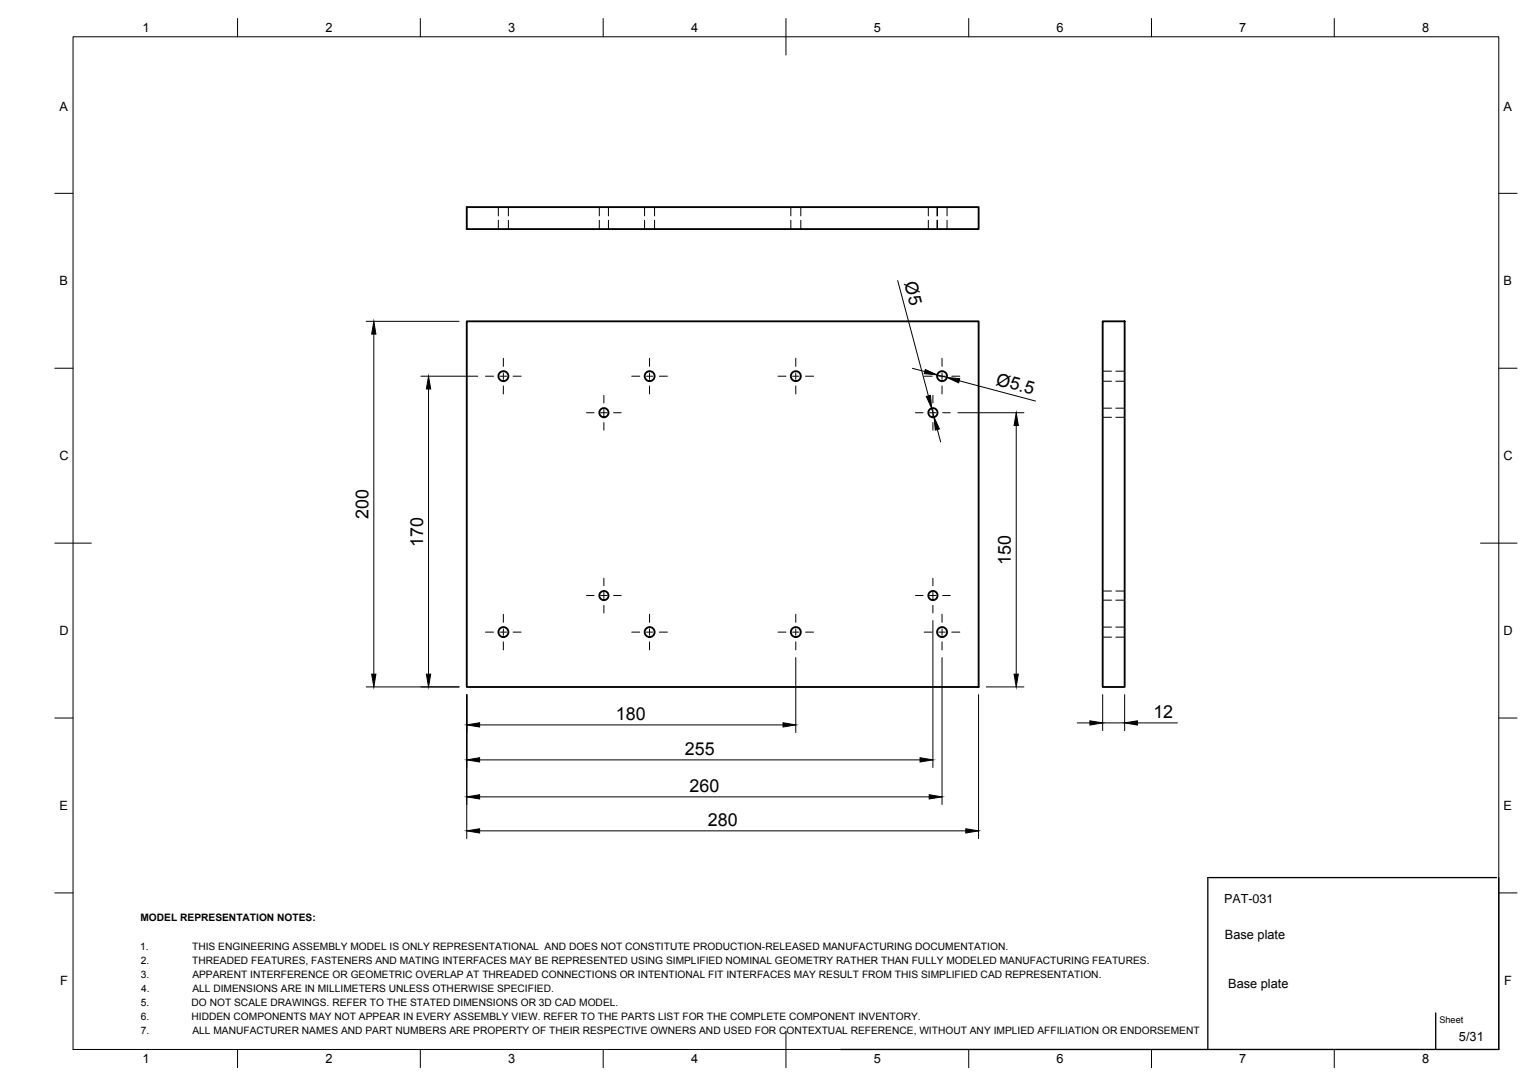
ISO-10303-21;
HEADER;
/* Generated by software containing ST-Developer
 * from STEP Tools, Inc. (www.steptools.com) 
 */

FILE_DESCRIPTION(
/* description */ ('Double-row support with tensioned shaft'),
/* implementation_level */ '2;1');

FILE_NAME(
/* name */ 'Base plate.step',
/* time_stamp */ '2026-10-27T10:50:35-07:00',
/* author */ (''),
/* organization */ (''),
/* preprocessor_version */ 'ST-DEVELOPER v20.2',
/* originating_system */ 'Autodesk Translation Framework v15.17.0.0',
/* authorisation */ '');

FILE_SCHEMA (('AUTOMOTIVE_DESIGN { 1 0 10303 214 3 1 1 }'));
ENDSEC;

DATA;
#10=MECHANICAL_DESIGN_GEOMETRIC_PRESENTATION_REPRESENTATION('',(#479),#11559);
#415=SHAPE_REPRESENTATION_RELATIONSHIP('SRR','None',#11723,#447);
#447=ADVANCED_BREP_SHAPE_REPRESENTATION('',(#512),#11525);
#479=STYLED_ITEM('',(#11946),#512);
#512=MANIFOLD_SOLID_BREP('Body1',#6324);
#542=FACE_BOUND('',#1278,.T.);
#543=FACE_BOUND('',#1279,.T.);
#544=FACE_BOUND('',#1280,.T.);
#545=FACE_BOUND('',#1281,.T.);
#546=FACE_BOUND('',#1282,.T.);
#547=FACE_BOUND('',#1283,.T.);
#548=FACE_BOUND('',#1284,.T.);
#549=FACE_BOUND('',#1285,.T.);
#550=FACE_BOUND('',#1286,.T.);
#551=FACE_BOUND('',#1287,.T.);
#552=FACE_BOUND('',#1288,.T.);
#553=FACE_BOUND('',#1289,.T.);
#554=FACE_BOUND('',#1291,.T.);
#555=FACE_BOUND('',#1292,.T.);
#556=FACE_BOUND('',#1293,.T.);
#557=FACE_BOUND('',#1294,.T.);
#558=FACE_BOUND('',#1295,.T.);
#559=FACE_BOUND('',#1296,.T.);
#560=FACE_BOUND('',#1297,.T.);
#561=FACE_BOUND('',#1298,.T.);
#562=FACE_BOUND('',#1299,.T.);
#563=FACE_BOUND('',#1300,.T.);
#564=FACE_BOUND('',#1301,.T.);
#565=FACE_BOUND('',#1302,.T.);
#679=PLANE('',#6752);
#680=PLANE('',#6753);
#681=PLANE('',#6754);
#682=PLANE('',#6755);
#683=PLANE('',#6756);
#684=PLANE('',#6757);
#917=FACE_OUTER_BOUND('',#1261,.T.);
#918=FACE_OUTER_BOUND('',#1262,.T.);
#919=FACE_OUTER_BOUND('',#1263,.T.);
#920=FACE_OUTER_BOUND('',#1264,.T.);
#921=FACE_OUTER_BOUND('',#1265,.T.);
#922=FACE_OUTER_BOUND('',#1266,.T.);
#923=FACE_OUTER_BOUND('',#1267,.T.);
#924=FACE_OUTER_BOUND('',#1268,.T.);
#925=FACE_OUTER_BOUND('',#1269,.T.);
#926=FACE_OUTER_BOUND('',#1270,.T.);
#927=FACE_OUTER_BOUND('',#1271,.T.);
#928=FACE_OUTER_BOUND('',#1272,.T.);
#929=FACE_OUTER_BOUND('',#1273,.T.);
#930=FACE_OUTER_BOUND('',#1274,.T.);
#931=FACE_OUTER_BOUND('',#1275,.T.);
#932=FACE_OUTER_BOUND('',#1276,.T.);
#933=FACE_OUTER_BOUND('',#1277,.T.);
#934=FACE_OUTER_BOUND('',#1290,.T.);
#1261=EDGE_LOOP('',(#4330,#4331,#4332,#4333));
#1262=EDGE_LOOP('',(#4334,#4335,#4336,#4337));
#1263=EDGE_LOOP('',(#4338,#4339,#4340,#4341));
#1264=EDGE_LOOP('',(#4342,#4343,#4344,#4345));
#1265=EDGE_LOOP('',(#4346,#4347,#4348,#4349));
#1266=EDGE_LOOP('',(#4350,#4351,#4352,#4353));
#1267=EDGE_LOOP('',(#4354,#4355,#4356,#4357));
#1268=EDGE_LOOP('',(#4358,#4359,#4360,#4361));
#1269=EDGE_LOOP('',(#4362,#4363,#4364,#4365));
#1270=EDGE_LOOP('',(#4366,#4367,#4368,#4369));
#1271=EDGE_LOOP('',(#4370,#4371,#4372,#4373));
#1272=EDGE_LOOP('',(#4374,#4375,#4376,#4377));
#1273=EDGE_LOOP('',(#4378,#4379,#4380,#4381));
#1274=EDGE_LOOP('',(#4382,#4383,#4384,#4385));
#1275=EDGE_LOOP('',(#4386,#4387,#4388,#4389));
#1276=EDGE_LOOP('',(#4390,#4391,#4392,#4393));
#1277=EDGE_LOOP('',(#4394,#4395,#4396,#4397));
#1278=EDGE_LOOP('',(#4398));
#1279=EDGE_LOOP('',(#4399));
#1280=EDGE_LOOP('',(#4400));
#1281=EDGE_LOOP('',(#4401));
#1282=EDGE_LOOP('',(#4402));
#1283=EDGE_LOOP('',(#4403));
#1284=EDGE_LOOP('',(#4404));
#1285=EDGE_LOOP('',(#4405));
#1286=EDGE_LOOP('',(#4406));
#1287=EDGE_LOOP('',(#4407));
#1288=EDGE_LOOP('',(#4408));
#1289=EDGE_LOOP('',(#4409));
#1290=EDGE_LOOP('',(#4410,#4411,#4412,#4413));
#1291=EDGE_LOOP('',(#4414));
#1292=EDGE_LOOP('',(#4415));
#1293=EDGE_LOOP('',(#4416));
#1294=EDGE_LOOP('',(#4417));
#1295=EDGE_LOOP('',(#4418));
#1296=EDGE_LOOP('',(#4419));
#1297=EDGE_LOOP('',(#4420));
#1298=EDGE_LOOP('',(#4421));
#1299=EDGE_LOOP('',(#4422));
#1300=EDGE_LOOP('',(#4423));
#1301=EDGE_LOOP('',(#4424));
#1302=EDGE_LOOP('',(#4425));
#1742=LINE('',#9241,#2289);
#1743=LINE('',#9247,#2290);
#1744=LINE('',#9253,#2291);
#1745=LINE('',#9259,#2292);
#1746=LINE('',#9265,#2293);
#1747=LINE('',#9271,#2294);
#1748=LINE('',#9277,#2295);
#1749=LINE('',#9283,#2296);
#1750=LINE('',#9289,#2297);
#1751=LINE('',#9295,#2298);
#1752=LINE('',#9301,#2299);
#1753=LINE('',#9307,#2300);
#1754=LINE('',#9312,#2301);
#1755=LINE('',#9314,#2302);
#1756=LINE('',#9316,#2303);
#1757=LINE('',#9317,#2304);
#1758=LINE('',#9320,#2305);
#1759=LINE('',#9322,#2306);
#1760=LINE('',#9323,#2307);
#1761=LINE('',#9326,#2308);
#1762=LINE('',#9328,#2309);
#1763=LINE('',#9329,#2310);
#1764=LINE('',#9331,#2311);
#1765=LINE('',#9332,#2312);
#2289=VECTOR('',#7381,0.25);
#2290=VECTOR('',#7388,0.25);
#2291=VECTOR('',#7395,0.25);
#2292=VECTOR('',#7402,0.25);
#2293=VECTOR('',#7409,0.275);
#2294=VECTOR('',#7416,0.275);
#2295=VECTOR('',#7423,0.275);
#2296=VECTOR('',#7430,0.275);
#2297=VECTOR('',#7437,0.275);
#2298=VECTOR('',#7444,0.275);
#2299=VECTOR('',#7451,0.275);
#2300=VECTOR('',#7458,0.275);
#2301=VECTOR('',#7463,1.);
#2302=VECTOR('',#7464,1.);
#2303=VECTOR('',#7465,1.);
#2304=VECTOR('',#7466,1.);
#2305=VECTOR('',#7469,1.);
#2306=VECTOR('',#7470,1.);
#2307=VECTOR('',#7471,1.);
#2308=VECTOR('',#7474,1.);
#2309=VECTOR('',#7475,1.);
#2310=VECTOR('',#7476,1.);
#2311=VECTOR('',#7479,1.);
#2312=VECTOR('',#7480,1.);
#2836=CIRCLE('',#6717,0.25);
#2837=CIRCLE('',#6718,0.25);
#2838=CIRCLE('',#6720,0.25);
#2839=CIRCLE('',#6721,0.25);
#2840=CIRCLE('',#6723,0.25);
#2841=CIRCLE('',#6724,0.25);
#2842=CIRCLE('',#6726,0.25);
#2843=CIRCLE('',#6727,0.25);
#2844=CIRCLE('',#6729,0.275);
#2845=CIRCLE('',#6730,0.275);
#2846=CIRCLE('',#6732,0.275);
#2847=CIRCLE('',#6733,0.275);
#2848=CIRCLE('',#6735,0.275);
#2849=CIRCLE('',#6736,0.275);
#2850=CIRCLE('',#6738,0.275);
#2851=CIRCLE('',#6739,0.275);
#2852=CIRCLE('',#6741,0.275);
#2853=CIRCLE('',#6742,0.275);
#2854=CIRCLE('',#6744,0.275);
#2855=CIRCLE('',#6745,0.275);
#2856=CIRCLE('',#6747,0.275);
#2857=CIRCLE('',#6748,0.275);
#2858=CIRCLE('',#6750,0.275);
#2859=CIRCLE('',#6751,0.275);
#3027=VERTEX_POINT('',#9238);
#3028=VERTEX_POINT('',#9240);
#3029=VERTEX_POINT('',#9244);
#3030=VERTEX_POINT('',#9246);
#3031=VERTEX_POINT('',#9250);
#3032=VERTEX_POINT('',#9252);
#3033=VERTEX_POINT('',#9256);
#3034=VERTEX_POINT('',#9258);
#3035=VERTEX_POINT('',#9262);
#3036=VERTEX_POINT('',#9264);
#3037=VERTEX_POINT('',#9268);
#3038=VERTEX_POINT('',#9270);
#3039=VERTEX_POINT('',#9274);
#3040=VERTEX_POINT('',#9276);
#3041=VERTEX_POINT('',#9280);
#3042=VERTEX_POINT('',#9282);
#3043=VERTEX_POINT('',#9286);
#3044=VERTEX_POINT('',#9288);
#3045=VERTEX_POINT('',#9292);
#3046=VERTEX_POINT('',#9294);
#3047=VERTEX_POINT('',#9298);
#3048=VERTEX_POINT('',#9300);
#3049=VERTEX_POINT('',#9304);
#3050=VERTEX_POINT('',#9306);
#3051=VERTEX_POINT('',#9310);
#3052=VERTEX_POINT('',#9311);
#3053=VERTEX_POINT('',#9313);
#3054=VERTEX_POINT('',#9315);
#3055=VERTEX_POINT('',#9319);
#3056=VERTEX_POINT('',#9321);
#3057=VERTEX_POINT('',#9325);
#3058=VERTEX_POINT('',#9327);
#3550=EDGE_CURVE('',#3027,#3027,#2836,.T.);
#3551=EDGE_CURVE('',#3027,#3028,#1742,.T.);
#3552=EDGE_CURVE('',#3028,#3028,#2837,.T.);
#3553=EDGE_CURVE('',#3029,#3029,#2838,.T.);
#3554=EDGE_CURVE('',#3029,#3030,#1743,.T.);
#3555=EDGE_CURVE('',#3030,#3030,#2839,.T.);
#3556=EDGE_CURVE('',#3031,#3031,#2840,.T.);
#3557=EDGE_CURVE('',#3031,#3032,#1744,.T.);
#3558=EDGE_CURVE('',#3032,#3032,#2841,.T.);
#3559=EDGE_CURVE('',#3033,#3033,#2842,.T.);
#3560=EDGE_CURVE('',#3033,#3034,#1745,.T.);
#3561=EDGE_CURVE('',#3034,#3034,#2843,.T.);
#3562=EDGE_CURVE('',#3035,#3035,#2844,.T.);
#3563=EDGE_CURVE('',#3035,#3036,#1746,.T.);
#3564=EDGE_CURVE('',#3036,#3036,#2845,.T.);
#3565=EDGE_CURVE('',#3037,#3037,#2846,.T.);
#3566=EDGE_CURVE('',#3037,#3038,#1747,.T.);
#3567=EDGE_CURVE('',#3038,#3038,#2847,.T.);
#3568=EDGE_CURVE('',#3039,#3039,#2848,.T.);
#3569=EDGE_CURVE('',#3039,#3040,#1748,.T.);
#3570=EDGE_CURVE('',#3040,#3040,#2849,.T.);
#3571=EDGE_CURVE('',#3041,#3041,#2850,.T.);
#3572=EDGE_CURVE('',#3041,#3042,#1749,.T.);
#3573=EDGE_CURVE('',#3042,#3042,#2851,.T.);
#3574=EDGE_CURVE('',#3043,#3043,#2852,.T.);
#3575=EDGE_CURVE('',#3043,#3044,#1750,.T.);
#3576=EDGE_CURVE('',#3044,#3044,#2853,.T.);
#3577=EDGE_CURVE('',#3045,#3045,#2854,.T.);
#3578=EDGE_CURVE('',#3045,#3046,#1751,.T.);
#3579=EDGE_CURVE('',#3046,#3046,#2855,.T.);
#3580=EDGE_CURVE('',#3047,#3047,#2856,.T.);
#3581=EDGE_CURVE('',#3047,#3048,#1752,.T.);
#3582=EDGE_CURVE('',#3048,#3048,#2857,.T.);
#3583=EDGE_CURVE('',#3049,#3049,#2858,.T.);
#3584=EDGE_CURVE('',#3049,#3050,#1753,.T.);
#3585=EDGE_CURVE('',#3050,#3050,#2859,.T.);
#3586=EDGE_CURVE('',#3051,#3052,#1754,.T.);
#3587=EDGE_CURVE('',#3052,#3053,#1755,.T.);
#3588=EDGE_CURVE('',#3054,#3053,#1756,.T.);
#3589=EDGE_CURVE('',#3051,#3054,#1757,.T.);
#3590=EDGE_CURVE('',#3055,#3051,#1758,.T.);
#3591=EDGE_CURVE('',#3056,#3054,#1759,.T.);
#3592=EDGE_CURVE('',#3055,#3056,#1760,.T.);
#3593=EDGE_CURVE('',#3057,#3055,#1761,.T.);
#3594=EDGE_CURVE('',#3058,#3056,#1762,.T.);
#3595=EDGE_CURVE('',#3057,#3058,#1763,.T.);
#3596=EDGE_CURVE('',#3052,#3057,#1764,.T.);
#3597=EDGE_CURVE('',#3053,#3058,#1765,.T.);
#4330=ORIENTED_EDGE('',*,*,#3550,.F.);
#4331=ORIENTED_EDGE('',*,*,#3551,.T.);
#4332=ORIENTED_EDGE('',*,*,#3552,.F.);
#4333=ORIENTED_EDGE('',*,*,#3551,.F.);
#4334=ORIENTED_EDGE('',*,*,#3553,.F.);
#4335=ORIENTED_EDGE('',*,*,#3554,.T.);
#4336=ORIENTED_EDGE('',*,*,#3555,.F.);
#4337=ORIENTED_EDGE('',*,*,#3554,.F.);
#4338=ORIENTED_EDGE('',*,*,#3556,.F.);
#4339=ORIENTED_EDGE('',*,*,#3557,.T.);
#4340=ORIENTED_EDGE('',*,*,#3558,.F.);
#4341=ORIENTED_EDGE('',*,*,#3557,.F.);
#4342=ORIENTED_EDGE('',*,*,#3559,.F.);
#4343=ORIENTED_EDGE('',*,*,#3560,.T.);
#4344=ORIENTED_EDGE('',*,*,#3561,.F.);
#4345=ORIENTED_EDGE('',*,*,#3560,.F.);
#4346=ORIENTED_EDGE('',*,*,#3562,.F.);
#4347=ORIENTED_EDGE('',*,*,#3563,.T.);
#4348=ORIENTED_EDGE('',*,*,#3564,.F.);
#4349=ORIENTED_EDGE('',*,*,#3563,.F.);
#4350=ORIENTED_EDGE('',*,*,#3565,.F.);
#4351=ORIENTED_EDGE('',*,*,#3566,.T.);
#4352=ORIENTED_EDGE('',*,*,#3567,.F.);
#4353=ORIENTED_EDGE('',*,*,#3566,.F.);
#4354=ORIENTED_EDGE('',*,*,#3568,.F.);
#4355=ORIENTED_EDGE('',*,*,#3569,.T.);
#4356=ORIENTED_EDGE('',*,*,#3570,.F.);
#4357=ORIENTED_EDGE('',*,*,#3569,.F.);
#4358=ORIENTED_EDGE('',*,*,#3571,.F.);
#4359=ORIENTED_EDGE('',*,*,#3572,.T.);
#4360=ORIENTED_EDGE('',*,*,#3573,.F.);
#4361=ORIENTED_EDGE('',*,*,#3572,.F.);
#4362=ORIENTED_EDGE('',*,*,#3574,.F.);
#4363=ORIENTED_EDGE('',*,*,#3575,.T.);
#4364=ORIENTED_EDGE('',*,*,#3576,.F.);
#4365=ORIENTED_EDGE('',*,*,#3575,.F.);
#4366=ORIENTED_EDGE('',*,*,#3577,.F.);
#4367=ORIENTED_EDGE('',*,*,#3578,.T.);
#4368=ORIENTED_EDGE('',*,*,#3579,.F.);
#4369=ORIENTED_EDGE('',*,*,#3578,.F.);
#4370=ORIENTED_EDGE('',*,*,#3580,.F.);
#4371=ORIENTED_EDGE('',*,*,#3581,.T.);
#4372=ORIENTED_EDGE('',*,*,#3582,.F.);
#4373=ORIENTED_EDGE('',*,*,#3581,.F.);
#4374=ORIENTED_EDGE('',*,*,#3583,.F.);
#4375=ORIENTED_EDGE('',*,*,#3584,.T.);
#4376=ORIENTED_EDGE('',*,*,#3585,.F.);
#4377=ORIENTED_EDGE('',*,*,#3584,.F.);
#4378=ORIENTED_EDGE('',*,*,#3586,.T.);
#4379=ORIENTED_EDGE('',*,*,#3587,.T.);
#4380=ORIENTED_EDGE('',*,*,#3588,.F.);
#4381=ORIENTED_EDGE('',*,*,#3589,.F.);
#4382=ORIENTED_EDGE('',*,*,#3590,.T.);
#4383=ORIENTED_EDGE('',*,*,#3589,.T.);
#4384=ORIENTED_EDGE('',*,*,#3591,.F.);
#4385=ORIENTED_EDGE('',*,*,#3592,.F.);
#4386=ORIENTED_EDGE('',*,*,#3593,.T.);
#4387=ORIENTED_EDGE('',*,*,#3592,.T.);
#4388=ORIENTED_EDGE('',*,*,#3594,.F.);
#4389=ORIENTED_EDGE('',*,*,#3595,.F.);
#4390=ORIENTED_EDGE('',*,*,#3596,.T.);
#4391=ORIENTED_EDGE('',*,*,#3595,.T.);
#4392=ORIENTED_EDGE('',*,*,#3597,.F.);
#4393=ORIENTED_EDGE('',*,*,#3587,.F.);
#4394=ORIENTED_EDGE('',*,*,#3597,.T.);
#4395=ORIENTED_EDGE('',*,*,#3594,.T.);
#4396=ORIENTED_EDGE('',*,*,#3591,.T.);
#4397=ORIENTED_EDGE('',*,*,#3588,.T.);
#4398=ORIENTED_EDGE('',*,*,#3558,.T.);
#4399=ORIENTED_EDGE('',*,*,#3561,.T.);
#4400=ORIENTED_EDGE('',*,*,#3585,.T.);
#4401=ORIENTED_EDGE('',*,*,#3582,.T.);
#4402=ORIENTED_EDGE('',*,*,#3579,.T.);
#4403=ORIENTED_EDGE('',*,*,#3576,.T.);
#4404=ORIENTED_EDGE('',*,*,#3573,.T.);
#4405=ORIENTED_EDGE('',*,*,#3570,.T.);
#4406=ORIENTED_EDGE('',*,*,#3567,.T.);
#4407=ORIENTED_EDGE('',*,*,#3564,.T.);
#4408=ORIENTED_EDGE('',*,*,#3555,.T.);
#4409=ORIENTED_EDGE('',*,*,#3552,.T.);
#4410=ORIENTED_EDGE('',*,*,#3596,.F.);
#4411=ORIENTED_EDGE('',*,*,#3586,.F.);
#4412=ORIENTED_EDGE('',*,*,#3590,.F.);
#4413=ORIENTED_EDGE('',*,*,#3593,.F.);
#4414=ORIENTED_EDGE('',*,*,#3556,.T.);
#4415=ORIENTED_EDGE('',*,*,#3559,.T.);
#4416=ORIENTED_EDGE('',*,*,#3583,.T.);
#4417=ORIENTED_EDGE('',*,*,#3580,.T.);
#4418=ORIENTED_EDGE('',*,*,#3577,.T.);
#4419=ORIENTED_EDGE('',*,*,#3574,.T.);
#4420=ORIENTED_EDGE('',*,*,#3571,.T.);
#4421=ORIENTED_EDGE('',*,*,#3568,.T.);
#4422=ORIENTED_EDGE('',*,*,#3565,.T.);
#4423=ORIENTED_EDGE('',*,*,#3562,.T.);
#4424=ORIENTED_EDGE('',*,*,#3553,.T.);
#4425=ORIENTED_EDGE('',*,*,#3550,.T.);
#5890=CYLINDRICAL_SURFACE('',#6716,0.25);
#5891=CYLINDRICAL_SURFACE('',#6719,0.25);
#5892=CYLINDRICAL_SURFACE('',#6722,0.25);
#5893=CYLINDRICAL_SURFACE('',#6725,0.25);
#5894=CYLINDRICAL_SURFACE('',#6728,0.275);
#5895=CYLINDRICAL_SURFACE('',#6731,0.275);
#5896=CYLINDRICAL_SURFACE('',#6734,0.275);
#5897=CYLINDRICAL_SURFACE('',#6737,0.275);
#5898=CYLINDRICAL_SURFACE('',#6740,0.275);
#5899=CYLINDRICAL_SURFACE('',#6743,0.275);
#5900=CYLINDRICAL_SURFACE('',#6746,0.275);
#5901=CYLINDRICAL_SURFACE('',#6749,0.275);
#5980=ADVANCED_FACE('',(#917),#5890,.F.);
#5981=ADVANCED_FACE('',(#918),#5891,.F.);
#5982=ADVANCED_FACE('',(#919),#5892,.F.);
#5983=ADVANCED_FACE('',(#920),#5893,.F.);
#5984=ADVANCED_FACE('',(#921),#5894,.F.);
#5985=ADVANCED_FACE('',(#922),#5895,.F.);
#5986=ADVANCED_FACE('',(#923),#5896,.F.);
#5987=ADVANCED_FACE('',(#924),#5897,.F.);
#5988=ADVANCED_FACE('',(#925),#5898,.F.);
#5989=ADVANCED_FACE('',(#926),#5899,.F.);
#5990=ADVANCED_FACE('',(#927),#5900,.F.);
#5991=ADVANCED_FACE('',(#928),#5901,.F.);
#5992=ADVANCED_FACE('',(#929),#679,.T.);
#5993=ADVANCED_FACE('',(#930),#680,.T.);
#5994=ADVANCED_FACE('',(#931),#681,.T.);
#5995=ADVANCED_FACE('',(#932),#682,.T.);
#5996=ADVANCED_FACE('',(#933,#542,#543,#544,#545,#546,#547,#548,#549,#550,
#551,#552,#553),#683,.T.);
#5997=ADVANCED_FACE('',(#934,#554,#555,#556,#557,#558,#559,#560,#561,#562,
#563,#564,#565),#684,.F.);
#6324=CLOSED_SHELL('',(#5980,#5981,#5982,#5983,#5984,#5985,#5986,#5987,
#5988,#5989,#5990,#5991,#5992,#5993,#5994,#5995,#5996,#5997));
#6715=AXIS2_PLACEMENT_3D('',#9236,#7375,#7376);
#6716=AXIS2_PLACEMENT_3D('',#9237,#7377,#7378);
#6717=AXIS2_PLACEMENT_3D('',#9239,#7379,#7380);
#6718=AXIS2_PLACEMENT_3D('',#9242,#7382,#7383);
#6719=AXIS2_PLACEMENT_3D('',#9243,#7384,#7385);
#6720=AXIS2_PLACEMENT_3D('',#9245,#7386,#7387);
#6721=AXIS2_PLACEMENT_3D('',#9248,#7389,#7390);
#6722=AXIS2_PLACEMENT_3D('',#9249,#7391,#7392);
#6723=AXIS2_PLACEMENT_3D('',#9251,#7393,#7394);
#6724=AXIS2_PLACEMENT_3D('',#9254,#7396,#7397);
#6725=AXIS2_PLACEMENT_3D('',#9255,#7398,#7399);
#6726=AXIS2_PLACEMENT_3D('',#9257,#7400,#7401);
#6727=AXIS2_PLACEMENT_3D('',#9260,#7403,#7404);
#6728=AXIS2_PLACEMENT_3D('',#9261,#7405,#7406);
#6729=AXIS2_PLACEMENT_3D('',#9263,#7407,#7408);
#6730=AXIS2_PLACEMENT_3D('',#9266,#7410,#7411);
#6731=AXIS2_PLACEMENT_3D('',#9267,#7412,#7413);
#6732=AXIS2_PLACEMENT_3D('',#9269,#7414,#7415);
#6733=AXIS2_PLACEMENT_3D('',#9272,#7417,#7418);
#6734=AXIS2_PLACEMENT_3D('',#9273,#7419,#7420);
#6735=AXIS2_PLACEMENT_3D('',#9275,#7421,#7422);
#6736=AXIS2_PLACEMENT_3D('',#9278,#7424,#7425);
#6737=AXIS2_PLACEMENT_3D('',#9279,#7426,#7427);
#6738=AXIS2_PLACEMENT_3D('',#9281,#7428,#7429);
#6739=AXIS2_PLACEMENT_3D('',#9284,#7431,#7432);
#6740=AXIS2_PLACEMENT_3D('',#9285,#7433,#7434);
#6741=AXIS2_PLACEMENT_3D('',#9287,#7435,#7436);
#6742=AXIS2_PLACEMENT_3D('',#9290,#7438,#7439);
#6743=AXIS2_PLACEMENT_3D('',#9291,#7440,#7441);
#6744=AXIS2_PLACEMENT_3D('',#9293,#7442,#7443);
#6745=AXIS2_PLACEMENT_3D('',#9296,#7445,#7446);
#6746=AXIS2_PLACEMENT_3D('',#9297,#7447,#7448);
#6747=AXIS2_PLACEMENT_3D('',#9299,#7449,#7450);
#6748=AXIS2_PLACEMENT_3D('',#9302,#7452,#7453);
#6749=AXIS2_PLACEMENT_3D('',#9303,#7454,#7455);
#6750=AXIS2_PLACEMENT_3D('',#9305,#7456,#7457);
#6751=AXIS2_PLACEMENT_3D('',#9308,#7459,#7460);
#6752=AXIS2_PLACEMENT_3D('',#9309,#7461,#7462);
#6753=AXIS2_PLACEMENT_3D('',#9318,#7467,#7468);
#6754=AXIS2_PLACEMENT_3D('',#9324,#7472,#7473);
#6755=AXIS2_PLACEMENT_3D('',#9330,#7477,#7478);
#6756=AXIS2_PLACEMENT_3D('',#9333,#7481,#7482);
#6757=AXIS2_PLACEMENT_3D('',#9334,#7483,#7484);
#7375=DIRECTION('axis',(0.,0.,1.));
#7376=DIRECTION('refdir',(1.,0.,0.));
#7377=DIRECTION('center_axis',(0.,0.,1.));
#7378=DIRECTION('ref_axis',(1.,0.,0.));
#7379=DIRECTION('center_axis',(0.,0.,1.));
#7380=DIRECTION('ref_axis',(1.,0.,0.));
#7381=DIRECTION('',(0.,0.,1.));
#7382=DIRECTION('center_axis',(0.,0.,-1.));
#7383=DIRECTION('ref_axis',(1.,0.,0.));
#7384=DIRECTION('center_axis',(0.,0.,1.));
#7385=DIRECTION('ref_axis',(1.,0.,0.));
#7386=DIRECTION('center_axis',(0.,0.,1.));
#7387=DIRECTION('ref_axis',(1.,0.,0.));
#7388=DIRECTION('',(0.,0.,1.));
#7389=DIRECTION('center_axis',(0.,0.,-1.));
#7390=DIRECTION('ref_axis',(1.,0.,0.));
#7391=DIRECTION('center_axis',(0.,0.,1.));
#7392=DIRECTION('ref_axis',(1.,0.,0.));
#7393=DIRECTION('center_axis',(0.,0.,1.));
#7394=DIRECTION('ref_axis',(1.,0.,0.));
#7395=DIRECTION('',(0.,0.,1.));
#7396=DIRECTION('center_axis',(0.,0.,-1.));
#7397=DIRECTION('ref_axis',(1.,0.,0.));
#7398=DIRECTION('center_axis',(0.,0.,1.));
#7399=DIRECTION('ref_axis',(1.,0.,0.));
#7400=DIRECTION('center_axis',(0.,0.,1.));
#7401=DIRECTION('ref_axis',(1.,0.,0.));
#7402=DIRECTION('',(0.,0.,1.));
#7403=DIRECTION('center_axis',(0.,0.,-1.));
#7404=DIRECTION('ref_axis',(1.,0.,0.));
#7405=DIRECTION('center_axis',(0.,0.,1.));
#7406=DIRECTION('ref_axis',(1.,0.,0.));
#7407=DIRECTION('center_axis',(0.,0.,1.));
#7408=DIRECTION('ref_axis',(1.,0.,0.));
#7409=DIRECTION('',(0.,0.,1.));
#7410=DIRECTION('center_axis',(0.,0.,-1.));
#7411=DIRECTION('ref_axis',(1.,0.,0.));
#7412=DIRECTION('center_axis',(0.,0.,1.));
#7413=DIRECTION('ref_axis',(1.,0.,0.));
#7414=DIRECTION('center_axis',(0.,0.,1.));
#7415=DIRECTION('ref_axis',(1.,0.,0.));
#7416=DIRECTION('',(0.,0.,1.));
#7417=DIRECTION('center_axis',(0.,0.,-1.));
#7418=DIRECTION('ref_axis',(1.,0.,0.));
#7419=DIRECTION('center_axis',(0.,0.,1.));
#7420=DIRECTION('ref_axis',(1.,0.,0.));
#7421=DIRECTION('center_axis',(0.,0.,1.));
#7422=DIRECTION('ref_axis',(1.,0.,0.));
#7423=DIRECTION('',(0.,0.,1.));
#7424=DIRECTION('center_axis',(0.,0.,-1.));
#7425=DIRECTION('ref_axis',(1.,0.,0.));
#7426=DIRECTION('center_axis',(0.,0.,1.));
#7427=DIRECTION('ref_axis',(1.,0.,0.));
#7428=DIRECTION('center_axis',(0.,0.,1.));
#7429=DIRECTION('ref_axis',(1.,0.,0.));
#7430=DIRECTION('',(0.,0.,1.));
#7431=DIRECTION('center_axis',(0.,0.,-1.));
#7432=DIRECTION('ref_axis',(1.,0.,0.));
#7433=DIRECTION('center_axis',(0.,0.,1.));
#7434=DIRECTION('ref_axis',(1.,0.,0.));
#7435=DIRECTION('center_axis',(0.,0.,1.));
#7436=DIRECTION('ref_axis',(1.,0.,0.));
#7437=DIRECTION('',(0.,0.,1.));
#7438=DIRECTION('center_axis',(0.,0.,-1.));
#7439=DIRECTION('ref_axis',(1.,0.,0.));
#7440=DIRECTION('center_axis',(0.,0.,1.));
#7441=DIRECTION('ref_axis',(1.,0.,0.));
#7442=DIRECTION('center_axis',(0.,0.,1.));
#7443=DIRECTION('ref_axis',(1.,0.,0.));
#7444=DIRECTION('',(0.,0.,1.));
#7445=DIRECTION('center_axis',(0.,0.,-1.));
#7446=DIRECTION('ref_axis',(1.,0.,0.));
#7447=DIRECTION('center_axis',(0.,0.,1.));
#7448=DIRECTION('ref_axis',(1.,0.,0.));
#7449=DIRECTION('center_axis',(0.,0.,1.));
#7450=DIRECTION('ref_axis',(1.,0.,0.));
#7451=DIRECTION('',(0.,0.,1.));
#7452=DIRECTION('center_axis',(0.,0.,-1.));
#7453=DIRECTION('ref_axis',(1.,0.,0.));
#7454=DIRECTION('center_axis',(0.,0.,1.));
#7455=DIRECTION('ref_axis',(1.,0.,0.));
#7456=DIRECTION('center_axis',(0.,0.,1.));
#7457=DIRECTION('ref_axis',(1.,0.,0.));
#7458=DIRECTION('',(0.,0.,1.));
#7459=DIRECTION('center_axis',(0.,0.,-1.));
#7460=DIRECTION('ref_axis',(1.,0.,0.));
#7461=DIRECTION('center_axis',(0.,1.,0.));
#7462=DIRECTION('ref_axis',(-1.,0.,0.));
#7463=DIRECTION('',(-1.,0.,0.));
#7464=DIRECTION('',(0.,0.,1.));
#7465=DIRECTION('',(-1.,0.,0.));
#7466=DIRECTION('',(0.,0.,1.));
#7467=DIRECTION('center_axis',(1.,0.,0.));
#7468=DIRECTION('ref_axis',(0.,1.,0.));
#7469=DIRECTION('',(0.,1.,0.));
#7470=DIRECTION('',(0.,1.,0.));
#7471=DIRECTION('',(0.,0.,1.));
#7472=DIRECTION('center_axis',(0.,-1.,0.));
#7473=DIRECTION('ref_axis',(1.,0.,0.));
#7474=DIRECTION('',(1.,0.,0.));
#7475=DIRECTION('',(1.,0.,0.));
#7476=DIRECTION('',(0.,0.,1.));
#7477=DIRECTION('center_axis',(-1.,0.,0.));
#7478=DIRECTION('ref_axis',(0.,-1.,0.));
#7479=DIRECTION('',(0.,-1.,0.));
#7480=DIRECTION('',(0.,-1.,0.));
#7481=DIRECTION('center_axis',(0.,0.,1.));
#7482=DIRECTION('ref_axis',(1.,0.,0.));
#7483=DIRECTION('center_axis',(0.,0.,1.));
#7484=DIRECTION('ref_axis',(1.,0.,0.));
#9236=CARTESIAN_POINT('',(0.,0.,0.));
#9237=CARTESIAN_POINT('Origin',(-5.,15.5,1.9));
#9238=CARTESIAN_POINT('',(-5.25,15.5,2.));
#9239=CARTESIAN_POINT('Origin',(-5.,15.5,2.));
#9240=CARTESIAN_POINT('',(-5.25,15.5,3.2));
#9241=CARTESIAN_POINT('',(-5.25,15.5,1.9));
#9242=CARTESIAN_POINT('Origin',(-5.,15.5,3.2));
#9243=CARTESIAN_POINT('Origin',(5.,15.5,1.9));
#9244=CARTESIAN_POINT('',(4.75,15.5,2.));
#9245=CARTESIAN_POINT('Origin',(5.,15.5,2.));
#9246=CARTESIAN_POINT('',(4.75,15.5,3.2));
#9247=CARTESIAN_POINT('',(4.75,15.5,1.9));
#9248=CARTESIAN_POINT('Origin',(5.,15.5,3.2));
#9249=CARTESIAN_POINT('Origin',(-5.,-2.5,1.9));
#9250=CARTESIAN_POINT('',(-5.25,-2.5,2.));
#9251=CARTESIAN_POINT('Origin',(-5.,-2.5,2.));
#9252=CARTESIAN_POINT('',(-5.25,-2.5,3.2));
#9253=CARTESIAN_POINT('',(-5.25,-2.5,1.9));
#9254=CARTESIAN_POINT('Origin',(-5.,-2.5,3.2));
#9255=CARTESIAN_POINT('Origin',(5.,-2.5,1.9));
#9256=CARTESIAN_POINT('',(4.75,-2.5,2.));
#9257=CARTESIAN_POINT('Origin',(5.,-2.5,2.));
#9258=CARTESIAN_POINT('',(4.75,-2.5,3.2));
#9259=CARTESIAN_POINT('',(4.75,-2.5,1.9));
#9260=CARTESIAN_POINT('Origin',(5.,-2.5,3.2));
#9261=CARTESIAN_POINT('Origin',(7.,13.,1.9));
#9262=CARTESIAN_POINT('',(6.725,13.,2.));
#9263=CARTESIAN_POINT('Origin',(7.,13.,2.));
#9264=CARTESIAN_POINT('',(6.725,13.,3.2));
#9265=CARTESIAN_POINT('',(6.725,13.,1.9));
#9266=CARTESIAN_POINT('Origin',(7.,13.,3.2));
#9267=CARTESIAN_POINT('Origin',(7.,-3.,1.9));
#9268=CARTESIAN_POINT('',(6.725,-3.,2.));
#9269=CARTESIAN_POINT('Origin',(7.,-3.,2.));
#9270=CARTESIAN_POINT('',(6.725,-3.,3.2));
#9271=CARTESIAN_POINT('',(6.725,-3.,1.9));
#9272=CARTESIAN_POINT('Origin',(7.,-3.,3.2));
#9273=CARTESIAN_POINT('Origin',(-7.,21.,1.9));
#9274=CARTESIAN_POINT('',(-7.275,21.,2.));
#9275=CARTESIAN_POINT('Origin',(-7.,21.,2.));
#9276=CARTESIAN_POINT('',(-7.275,21.,3.2));
#9277=CARTESIAN_POINT('',(-7.275,21.,1.9));
#9278=CARTESIAN_POINT('Origin',(-7.,21.,3.2));
#9279=CARTESIAN_POINT('Origin',(-7.,5.,1.9));
#9280=CARTESIAN_POINT('',(-7.275,5.,2.));
#9281=CARTESIAN_POINT('Origin',(-7.,5.,2.));
#9282=CARTESIAN_POINT('',(-7.275,5.,3.2));
#9283=CARTESIAN_POINT('',(-7.275,5.,1.9));
#9284=CARTESIAN_POINT('Origin',(-7.,5.,3.2));
#9285=CARTESIAN_POINT('Origin',(-7.,13.,1.9));
#9286=CARTESIAN_POINT('',(-7.275,13.,2.));
#9287=CARTESIAN_POINT('Origin',(-7.,13.,2.));
#9288=CARTESIAN_POINT('',(-7.275,13.,3.2));
#9289=CARTESIAN_POINT('',(-7.275,13.,1.9));
#9290=CARTESIAN_POINT('Origin',(-7.,13.,3.2));
#9291=CARTESIAN_POINT('Origin',(-7.,-3.,1.9));
#9292=CARTESIAN_POINT('',(-7.275,-3.,2.));
#9293=CARTESIAN_POINT('Origin',(-7.,-3.,2.));
#9294=CARTESIAN_POINT('',(-7.275,-3.,3.2));
#9295=CARTESIAN_POINT('',(-7.275,-3.,1.9));
#9296=CARTESIAN_POINT('Origin',(-7.,-3.,3.2));
#9297=CARTESIAN_POINT('Origin',(7.,5.,1.9));
#9298=CARTESIAN_POINT('',(6.725,5.,2.));
#9299=CARTESIAN_POINT('Origin',(7.,5.,2.));
#9300=CARTESIAN_POINT('',(6.725,5.,3.2));
#9301=CARTESIAN_POINT('',(6.725,5.,1.9));
#9302=CARTESIAN_POINT('Origin',(7.,5.,3.2));
#9303=CARTESIAN_POINT('Origin',(7.,21.,1.9));
#9304=CARTESIAN_POINT('',(6.725,21.,2.));
#9305=CARTESIAN_POINT('Origin',(7.,21.,2.));
#9306=CARTESIAN_POINT('',(6.725,21.,3.2));
#9307=CARTESIAN_POINT('',(6.725,21.,1.9));
#9308=CARTESIAN_POINT('Origin',(7.,21.,3.2));
#9309=CARTESIAN_POINT('Origin',(10.,23.,2.));
#9310=CARTESIAN_POINT('',(10.,23.,2.));
#9311=CARTESIAN_POINT('',(-10.,23.,2.));
#9312=CARTESIAN_POINT('',(10.,23.,2.));
#9313=CARTESIAN_POINT('',(-10.,23.,3.2));
#9314=CARTESIAN_POINT('',(-10.,23.,2.));
#9315=CARTESIAN_POINT('',(10.,23.,3.2));
#9316=CARTESIAN_POINT('',(10.,23.,3.2));
#9317=CARTESIAN_POINT('',(10.,23.,2.));
#9318=CARTESIAN_POINT('Origin',(10.,-5.,2.));
#9319=CARTESIAN_POINT('',(10.,-5.,2.));
#9320=CARTESIAN_POINT('',(10.,-5.,2.));
#9321=CARTESIAN_POINT('',(10.,-5.,3.2));
#9322=CARTESIAN_POINT('',(10.,-5.,3.2));
#9323=CARTESIAN_POINT('',(10.,-5.,2.));
#9324=CARTESIAN_POINT('Origin',(-10.,-5.,2.));
#9325=CARTESIAN_POINT('',(-10.,-5.,2.));
#9326=CARTESIAN_POINT('',(-10.,-5.,2.));
#9327=CARTESIAN_POINT('',(-10.,-5.,3.2));
#9328=CARTESIAN_POINT('',(-10.,-5.,3.2));
#9329=CARTESIAN_POINT('',(-10.,-5.,2.));
#9330=CARTESIAN_POINT('Origin',(-10.,23.,2.));
#9331=CARTESIAN_POINT('',(-10.,23.,2.));
#9332=CARTESIAN_POINT('',(-10.,23.,3.2));
#9333=CARTESIAN_POINT('Origin',(0.,9.,3.2));
#9334=CARTESIAN_POINT('Origin',(0.,9.,2.));
#11488=UNCERTAINTY_MEASURE_WITH_UNIT(LENGTH_MEASURE(0.001),#11560,
'DISTANCE_ACCURACY_VALUE',
'Maximum model space distance between geometric entities at asserted c
onnectivities');
#11522=UNCERTAINTY_MEASURE_WITH_UNIT(LENGTH_MEASURE(0.001),#11560,
'DISTANCE_ACCURACY_VALUE',
'Maximum model space distance between geometric entities at asserted c
onnectivities');
#11525=(
GEOMETRIC_REPRESENTATION_CONTEXT(3)
GLOBAL_UNCERTAINTY_ASSIGNED_CONTEXT((#11488))
GLOBAL_UNIT_ASSIGNED_CONTEXT((#11560,#11562,#11563))
REPRESENTATION_CONTEXT('','3D')
);
#11559=(
GEOMETRIC_REPRESENTATION_CONTEXT(3)
GLOBAL_UNCERTAINTY_ASSIGNED_CONTEXT((#11522))
GLOBAL_UNIT_ASSIGNED_CONTEXT((#11560,#11562,#11563))
REPRESENTATION_CONTEXT('','3D')
);
#11560=(
LENGTH_UNIT()
NAMED_UNIT(*)
SI_UNIT(.CENTI.,.METRE.)
);
#11562=(
NAMED_UNIT(*)
PLANE_ANGLE_UNIT()
SI_UNIT($,.RADIAN.)
);
#11563=(
NAMED_UNIT(*)
SI_UNIT($,.STERADIAN.)
SOLID_ANGLE_UNIT()
);
#11566=SHAPE_DEFINITION_REPRESENTATION(#11602,#11723);
#11602=PRODUCT_DEFINITION_SHAPE('',$,#11760);
#11723=SHAPE_REPRESENTATION('',(#6715),#11525);
#11757=PRODUCT_DEFINITION_CONTEXT('part definition',#11867,'design');
#11760=PRODUCT_DEFINITION('Base plate','Base plate',#11796,#11757);
#11796=PRODUCT_DEFINITION_FORMATION('',$,#11871);
#11867=APPLICATION_CONTEXT(
'Core Data for Automotive Mechanical Design Process');
#11868=PRODUCT_CONTEXT('part definition',#11867,'mechanical');
#11871=PRODUCT('Base plate','Base plate','Base plate',(#11868));
#11940=COLOUR_RGB('Dark Blue',0.08,0.2,0.34);
#11941=FILL_AREA_STYLE_COLOUR('',#11940);
#11942=FILL_AREA_STYLE('',(#11941));
#11943=SURFACE_STYLE_FILL_AREA(#11942);
#11944=SURFACE_SIDE_STYLE('',(#11943));
#11945=SURFACE_STYLE_USAGE(.BOTH.,#11944);
#11946=PRESENTATION_STYLE_ASSIGNMENT((#11945));
ENDSEC;
END-ISO-10303-21;
